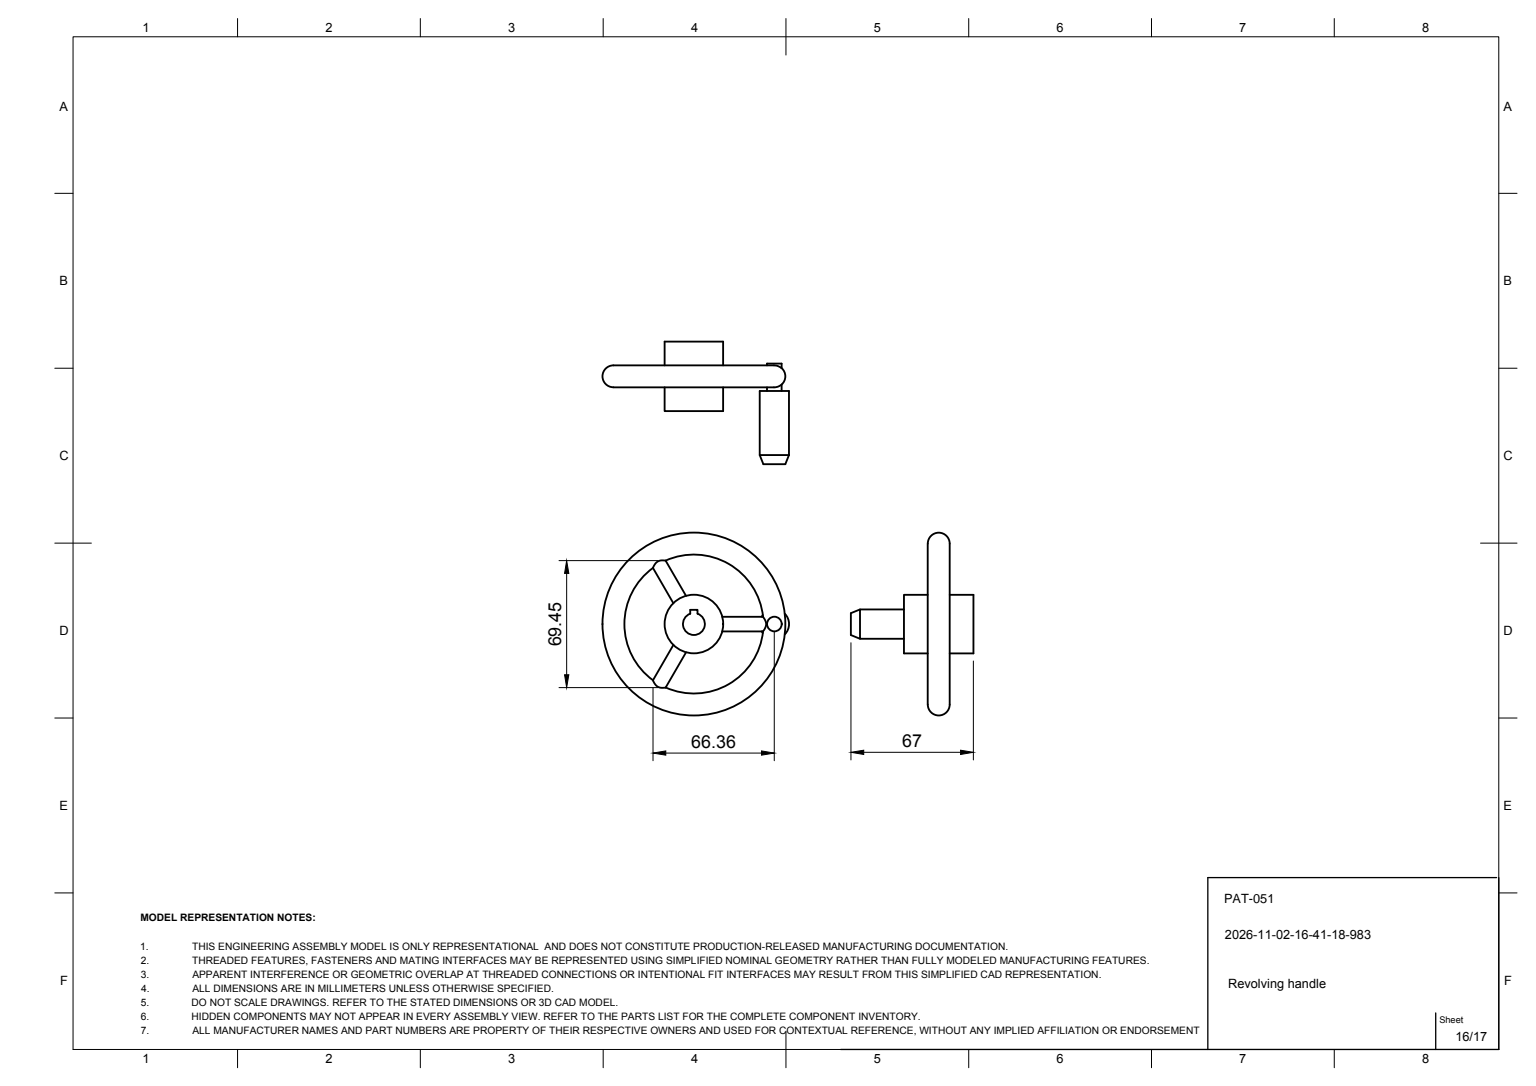
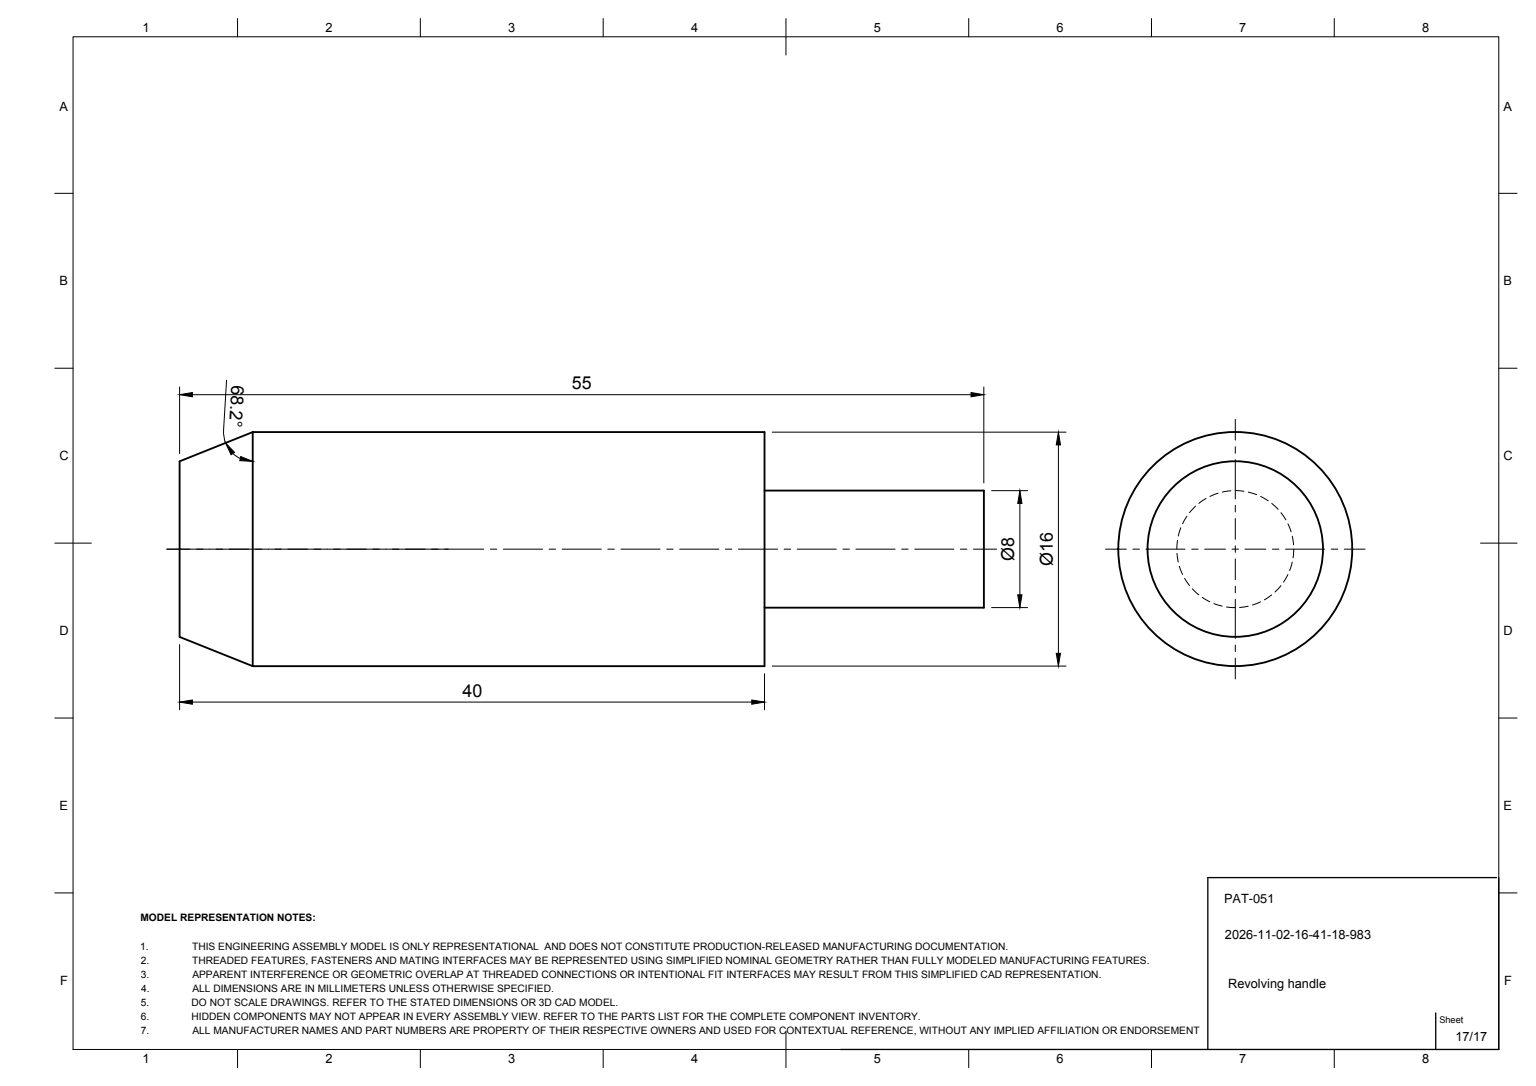
ISO-10303-21;
HEADER;
/* Generated by software containing ST-Developer
 * from STEP Tools, Inc. (www.steptools.com) 
 */

FILE_DESCRIPTION(
/* description */ ('Hand-crank flanged shaft unit'),
/* implementation_level */ '2;1');

FILE_NAME(
/* name */ 'Revolving handle.step',
/* time_stamp */ '2026-10-27T18:35:45-07:00',
/* author */ (''),
/* organization */ (''),
/* preprocessor_version */ 'ST-DEVELOPER v20.2',
/* originating_system */ 'Autodesk Translation Framework v15.17.0.0',
/* authorisation */ '');

FILE_SCHEMA (('AUTOMOTIVE_DESIGN { 1 0 10303 214 3 1 1 }'));
ENDSEC;

DATA;
#10=MECHANICAL_DESIGN_GEOMETRIC_PRESENTATION_REPRESENTATION('',(#294),#6805);
#17=CONICAL_SURFACE('',#3823,0.699999999999999,0.380506377112365);
#253=SHAPE_REPRESENTATION_RELATIONSHIP('SRR','None',#6917,#273);
#273=ADVANCED_BREP_SHAPE_REPRESENTATION('',(#314),#6800);
#294=STYLED_ITEM('',(#7084),#314);
#314=MANIFOLD_SOLID_BREP('Body1',#3336);
#395=FACE_BOUND('',#906,.T.);
#479=PLANE('',#3821);
#480=PLANE('',#3827);
#481=PLANE('',#3831);
#639=FACE_OUTER_BOUND('',#902,.T.);
#640=FACE_OUTER_BOUND('',#903,.T.);
#641=FACE_OUTER_BOUND('',#904,.T.);
#642=FACE_OUTER_BOUND('',#905,.T.);
#643=FACE_OUTER_BOUND('',#907,.T.);
#644=FACE_OUTER_BOUND('',#908,.T.);
#902=EDGE_LOOP('',(#2773));
#903=EDGE_LOOP('',(#2774,#2775,#2776,#2777));
#904=EDGE_LOOP('',(#2778,#2779,#2780,#2781));
#905=EDGE_LOOP('',(#2782));
#906=EDGE_LOOP('',(#2783));
#907=EDGE_LOOP('',(#2784,#2785,#2786,#2787));
#908=EDGE_LOOP('',(#2788));
#1122=LINE('',#5960,#1350);
#1123=LINE('',#5964,#1351);
#1124=LINE('',#5971,#1352);
#1350=VECTOR('',#4623,0.699999999999999);
#1351=VECTOR('',#4628,0.8);
#1352=VECTOR('',#4637,0.399999999999999);
#1533=CIRCLE('',#3822,0.6);
#1534=CIRCLE('',#3824,0.8);
#1535=CIRCLE('',#3826,0.8);
#1536=CIRCLE('',#3828,0.399999999999999);
#1537=CIRCLE('',#3830,0.399999999999999);
#1749=VERTEX_POINT('',#5955);
#1750=VERTEX_POINT('',#5958);
#1751=VERTEX_POINT('',#5962);
#1752=VERTEX_POINT('',#5966);
#1753=VERTEX_POINT('',#5969);
#2104=EDGE_CURVE('',#1749,#1749,#1533,.T.);
#2105=EDGE_CURVE('',#1750,#1750,#1534,.T.);
#2106=EDGE_CURVE('',#1750,#1749,#1122,.T.);
#2107=EDGE_CURVE('',#1751,#1751,#1535,.T.);
#2108=EDGE_CURVE('',#1751,#1750,#1123,.T.);
#2109=EDGE_CURVE('',#1752,#1752,#1536,.T.);
#2110=EDGE_CURVE('',#1753,#1753,#1537,.T.);
#2111=EDGE_CURVE('',#1753,#1752,#1124,.T.);
#2773=ORIENTED_EDGE('',*,*,#2104,.F.);
#2774=ORIENTED_EDGE('',*,*,#2105,.F.);
#2775=ORIENTED_EDGE('',*,*,#2106,.T.);
#2776=ORIENTED_EDGE('',*,*,#2104,.T.);
#2777=ORIENTED_EDGE('',*,*,#2106,.F.);
#2778=ORIENTED_EDGE('',*,*,#2107,.F.);
#2779=ORIENTED_EDGE('',*,*,#2108,.T.);
#2780=ORIENTED_EDGE('',*,*,#2105,.T.);
#2781=ORIENTED_EDGE('',*,*,#2108,.F.);
#2782=ORIENTED_EDGE('',*,*,#2107,.T.);
#2783=ORIENTED_EDGE('',*,*,#2109,.F.);
#2784=ORIENTED_EDGE('',*,*,#2110,.F.);
#2785=ORIENTED_EDGE('',*,*,#2111,.T.);
#2786=ORIENTED_EDGE('',*,*,#2109,.T.);
#2787=ORIENTED_EDGE('',*,*,#2111,.F.);
#2788=ORIENTED_EDGE('',*,*,#2110,.T.);
#3116=CYLINDRICAL_SURFACE('',#3825,0.8);
#3117=CYLINDRICAL_SURFACE('',#3829,0.399999999999999);
#3256=ADVANCED_FACE('',(#639),#479,.T.);
#3257=ADVANCED_FACE('',(#640),#17,.T.);
#3258=ADVANCED_FACE('',(#641),#3116,.T.);
#3259=ADVANCED_FACE('',(#642,#395),#480,.T.);
#3260=ADVANCED_FACE('',(#643),#3117,.T.);
#3261=ADVANCED_FACE('',(#644),#481,.T.);
#3336=CLOSED_SHELL('',(#3256,#3257,#3258,#3259,#3260,#3261));
#3820=AXIS2_PLACEMENT_3D('',#5953,#4613,#4614);
#3821=AXIS2_PLACEMENT_3D('',#5954,#4615,#4616);
#3822=AXIS2_PLACEMENT_3D('',#5956,#4617,#4618);
#3823=AXIS2_PLACEMENT_3D('',#5957,#4619,#4620);
#3824=AXIS2_PLACEMENT_3D('',#5959,#4621,#4622);
#3825=AXIS2_PLACEMENT_3D('',#5961,#4624,#4625);
#3826=AXIS2_PLACEMENT_3D('',#5963,#4626,#4627);
#3827=AXIS2_PLACEMENT_3D('',#5965,#4629,#4630);
#3828=AXIS2_PLACEMENT_3D('',#5967,#4631,#4632);
#3829=AXIS2_PLACEMENT_3D('',#5968,#4633,#4634);
#3830=AXIS2_PLACEMENT_3D('',#5970,#4635,#4636);
#3831=AXIS2_PLACEMENT_3D('',#5972,#4638,#4639);
#4613=DIRECTION('axis',(0.,0.,1.));
#4614=DIRECTION('refdir',(1.,0.,0.));
#4615=DIRECTION('center_axis',(0.,1.,0.));
#4616=DIRECTION('ref_axis',(0.,0.,1.));
#4617=DIRECTION('center_axis',(0.,-1.,0.));
#4618=DIRECTION('ref_axis',(1.,0.,0.));
#4619=DIRECTION('center_axis',(0.,-1.,0.));
#4620=DIRECTION('ref_axis',(1.,0.,0.));
#4621=DIRECTION('center_axis',(0.,-1.,0.));
#4622=DIRECTION('ref_axis',(1.,0.,0.));
#4623=DIRECTION('',(0.371390676354104,0.928476690885259,4.54822403030224E-17));
#4624=DIRECTION('center_axis',(0.,-1.,0.));
#4625=DIRECTION('ref_axis',(1.,0.,0.));
#4626=DIRECTION('center_axis',(0.,-1.,0.));
#4627=DIRECTION('ref_axis',(1.,0.,0.));
#4628=DIRECTION('',(0.,1.,0.));
#4629=DIRECTION('center_axis',(0.,-1.,0.));
#4630=DIRECTION('ref_axis',(0.,0.,-1.));
#4631=DIRECTION('center_axis',(0.,-1.,0.));
#4632=DIRECTION('ref_axis',(1.,0.,0.));
#4633=DIRECTION('center_axis',(0.,-1.,0.));
#4634=DIRECTION('ref_axis',(1.,0.,0.));
#4635=DIRECTION('center_axis',(0.,-1.,0.));
#4636=DIRECTION('ref_axis',(1.,0.,0.));
#4637=DIRECTION('',(0.,1.,0.));
#4638=DIRECTION('center_axis',(0.,-1.,0.));
#4639=DIRECTION('ref_axis',(0.,0.,-1.));
#5953=CARTESIAN_POINT('',(0.,0.,0.));
#5954=CARTESIAN_POINT('Origin',(5.,4.8,0.));
#5955=CARTESIAN_POINT('',(3.8,4.8,-7.34788079488411E-17));
#5956=CARTESIAN_POINT('Origin',(4.4,4.8,0.));
#5957=CARTESIAN_POINT('Origin',(4.4,4.55,0.));
#5958=CARTESIAN_POINT('',(3.6,4.3,-9.79717439317882E-17));
#5959=CARTESIAN_POINT('Origin',(4.4,4.3,0.));
#5960=CARTESIAN_POINT('',(3.7,4.55,-8.57252759403146E-17));
#5961=CARTESIAN_POINT('Origin',(4.4,2.55,0.));
#5962=CARTESIAN_POINT('',(3.6,0.8,-9.79717439317882E-17));
#5963=CARTESIAN_POINT('Origin',(4.4,0.8,0.));
#5964=CARTESIAN_POINT('',(3.6,2.55,-9.79717439317882E-17));
#5965=CARTESIAN_POINT('Origin',(4.8,0.8,0.));
#5966=CARTESIAN_POINT('',(4.,0.8,-4.89858719658941E-17));
#5967=CARTESIAN_POINT('Origin',(4.4,0.8,0.));
#5968=CARTESIAN_POINT('Origin',(4.4,0.05,0.));
#5969=CARTESIAN_POINT('',(4.,-0.7,-4.89858719658941E-17));
#5970=CARTESIAN_POINT('Origin',(4.4,-0.7,0.));
#5971=CARTESIAN_POINT('',(4.,0.05,-4.89858719658941E-17));
#5972=CARTESIAN_POINT('Origin',(4.4,-0.7,0.));
#6775=UNCERTAINTY_MEASURE_WITH_UNIT(LENGTH_MEASURE(0.001),#6806,
'DISTANCE_ACCURACY_VALUE',
'Maximum model space distance between geometric entities at asserted c
onnectivities');
#6780=UNCERTAINTY_MEASURE_WITH_UNIT(LENGTH_MEASURE(0.001),#6806,
'DISTANCE_ACCURACY_VALUE',
'Maximum model space distance between geometric entities at asserted c
onnectivities');
#6800=(
GEOMETRIC_REPRESENTATION_CONTEXT(3)
GLOBAL_UNCERTAINTY_ASSIGNED_CONTEXT((#6775))
GLOBAL_UNIT_ASSIGNED_CONTEXT((#6806,#6808,#6809))
REPRESENTATION_CONTEXT('','3D')
);
#6805=(
GEOMETRIC_REPRESENTATION_CONTEXT(3)
GLOBAL_UNCERTAINTY_ASSIGNED_CONTEXT((#6780))
GLOBAL_UNIT_ASSIGNED_CONTEXT((#6806,#6808,#6809))
REPRESENTATION_CONTEXT('','3D')
);
#6806=(
LENGTH_UNIT()
NAMED_UNIT(*)
SI_UNIT(.CENTI.,.METRE.)
);
#6808=(
NAMED_UNIT(*)
PLANE_ANGLE_UNIT()
SI_UNIT($,.RADIAN.)
);
#6809=(
NAMED_UNIT(*)
SI_UNIT($,.STERADIAN.)
SOLID_ANGLE_UNIT()
);
#6829=SHAPE_DEFINITION_REPRESENTATION(#6882,#6917);
#6882=PRODUCT_DEFINITION_SHAPE('',$,#6942);
#6917=SHAPE_REPRESENTATION('',(#3820),#6800);
#6922=PRODUCT_DEFINITION_CONTEXT('part definition',#6996,'design');
#6942=PRODUCT_DEFINITION('Revolving handle','Revolving handle',#6966,#6922);
#6966=PRODUCT_DEFINITION_FORMATION('',$,#7017);
#6996=APPLICATION_CONTEXT(
'Core Data for Automotive Mechanical Design Process');
#6997=PRODUCT_CONTEXT('part definition',#6996,'mechanical');
#7017=PRODUCT('Revolving handle','Revolving handle','Revolving handle',
(#6997));
#7078=COLOUR_RGB('Sky Blue',0.24,0.69,0.87);
#7079=FILL_AREA_STYLE_COLOUR('',#7078);
#7080=FILL_AREA_STYLE('',(#7079));
#7081=SURFACE_STYLE_FILL_AREA(#7080);
#7082=SURFACE_SIDE_STYLE('',(#7081));
#7083=SURFACE_STYLE_USAGE(.BOTH.,#7082);
#7084=PRESENTATION_STYLE_ASSIGNMENT((#7083));
ENDSEC;
END-ISO-10303-21;
